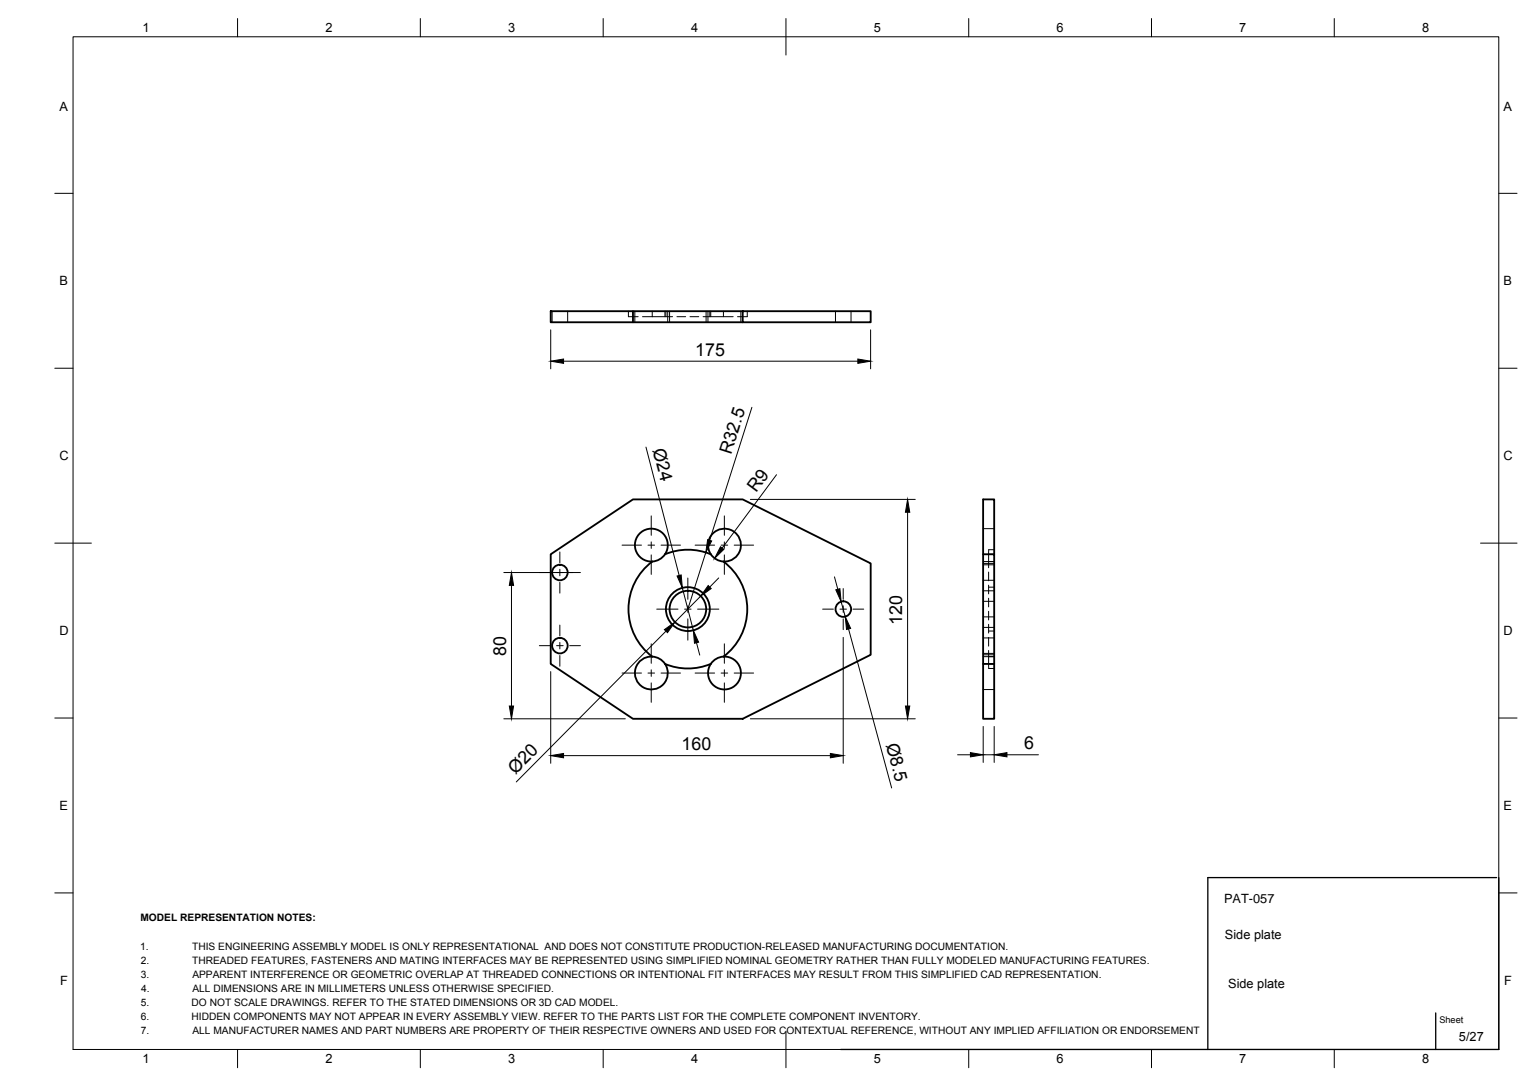
ISO-10303-21;
HEADER;
/* Generated by software containing ST-Developer
 * from STEP Tools, Inc. (www.steptools.com) 
 */

FILE_DESCRIPTION(
/* description */ ('Bearing-mounted hook block'),
/* implementation_level */ '2;1');

FILE_NAME(
/* name */ 'Side plate.step',
/* time_stamp */ '2026-10-28T22:30:11-07:00',
/* author */ (''),
/* organization */ (''),
/* preprocessor_version */ 'ST-DEVELOPER v20.2',
/* originating_system */ 'Autodesk Translation Framework v15.17.0.0',
/* authorisation */ '');

FILE_SCHEMA (('AUTOMOTIVE_DESIGN { 1 0 10303 214 3 1 1 }'));
ENDSEC;

DATA;
#10=MECHANICAL_DESIGN_GEOMETRIC_PRESENTATION_REPRESENTATION('',(#323),#7609);
#275=SHAPE_REPRESENTATION_RELATIONSHIP('SRR','None',#7722,#299);
#299=ADVANCED_BREP_SHAPE_REPRESENTATION('',(#355),#7582);
#323=STYLED_ITEM('',(#7924),#355);
#355=MANIFOLD_SOLID_BREP('Body1',#3919);
#384=LINE('',#6087,#614);
#385=LINE('',#6089,#615);
#386=LINE('',#6093,#616);
#387=LINE('',#6096,#617);
#388=LINE('',#6099,#618);
#389=LINE('',#6101,#619);
#390=LINE('',#6105,#620);
#391=LINE('',#6109,#621);
#392=LINE('',#6112,#622);
#393=LINE('',#6117,#623);
#394=LINE('',#6124,#624);
#395=LINE('',#6131,#625);
#396=LINE('',#6141,#626);
#397=LINE('',#6148,#627);
#398=LINE('',#6154,#628);
#399=LINE('',#6160,#629);
#400=LINE('',#6165,#630);
#401=LINE('',#6169,#631);
#402=LINE('',#6171,#632);
#403=LINE('',#6173,#633);
#404=LINE('',#6174,#634);
#405=LINE('',#6177,#635);
#406=LINE('',#6179,#636);
#407=LINE('',#6180,#637);
#408=LINE('',#6183,#638);
#409=LINE('',#6185,#639);
#410=LINE('',#6186,#640);
#411=LINE('',#6189,#641);
#412=LINE('',#6191,#642);
#413=LINE('',#6192,#643);
#414=LINE('',#6195,#644);
#415=LINE('',#6197,#645);
#416=LINE('',#6198,#646);
#417=LINE('',#6201,#647);
#418=LINE('',#6203,#648);
#419=LINE('',#6204,#649);
#420=LINE('',#6207,#650);
#421=LINE('',#6209,#651);
#422=LINE('',#6210,#652);
#423=LINE('',#6212,#653);
#424=LINE('',#6213,#654);
#614=VECTOR('',#4785,1.);
#615=VECTOR('',#4786,1.);
#616=VECTOR('',#4791,1.);
#617=VECTOR('',#4794,1.);
#618=VECTOR('',#4797,1.);
#619=VECTOR('',#4798,1.);
#620=VECTOR('',#4803,1.2);
#621=VECTOR('',#4808,1.);
#622=VECTOR('',#4811,1.);
#623=VECTOR('',#4816,0.9);
#624=VECTOR('',#4825,0.9);
#625=VECTOR('',#4834,0.9);
#626=VECTOR('',#4847,0.9);
#627=VECTOR('',#4856,0.425);
#628=VECTOR('',#4863,0.425);
#629=VECTOR('',#4870,0.425);
#630=VECTOR('',#4877,1.);
#631=VECTOR('',#4880,1.);
#632=VECTOR('',#4881,1.);
#633=VECTOR('',#4882,1.);
#634=VECTOR('',#4883,1.);
#635=VECTOR('',#4886,1.);
#636=VECTOR('',#4887,1.);
#637=VECTOR('',#4888,1.);
#638=VECTOR('',#4891,1.);
#639=VECTOR('',#4892,1.);
#640=VECTOR('',#4893,1.);
#641=VECTOR('',#4896,1.);
#642=VECTOR('',#4897,1.);
#643=VECTOR('',#4898,1.);
#644=VECTOR('',#4901,1.);
#645=VECTOR('',#4902,1.);
#646=VECTOR('',#4903,1.);
#647=VECTOR('',#4906,1.);
#648=VECTOR('',#4907,1.);
#649=VECTOR('',#4908,1.);
#650=VECTOR('',#4911,1.);
#651=VECTOR('',#4912,1.);
#652=VECTOR('',#4913,1.);
#653=VECTOR('',#4916,1.);
#654=VECTOR('',#4917,1.);
#844=CYLINDRICAL_SURFACE('',#4232,3.25);
#845=CYLINDRICAL_SURFACE('',#4234,3.25);
#846=CYLINDRICAL_SURFACE('',#4236,3.25);
#847=CYLINDRICAL_SURFACE('',#4238,1.2);
#848=CYLINDRICAL_SURFACE('',#4240,3.25);
#849=CYLINDRICAL_SURFACE('',#4242,0.9);
#850=CYLINDRICAL_SURFACE('',#4246,0.9);
#851=CYLINDRICAL_SURFACE('',#4250,0.9);
#852=CYLINDRICAL_SURFACE('',#4256,0.9);
#853=CYLINDRICAL_SURFACE('',#4260,0.425);
#854=CYLINDRICAL_SURFACE('',#4263,0.425);
#855=CYLINDRICAL_SURFACE('',#4266,0.425);
#856=CYLINDRICAL_SURFACE('',#4269,1.);
#921=FACE_BOUND('',#1238,.T.);
#922=FACE_BOUND('',#1248,.T.);
#923=FACE_BOUND('',#1263,.T.);
#924=FACE_BOUND('',#1264,.T.);
#925=FACE_BOUND('',#1265,.T.);
#926=FACE_BOUND('',#1266,.T.);
#927=FACE_BOUND('',#1268,.T.);
#928=FACE_BOUND('',#1269,.T.);
#929=FACE_BOUND('',#1270,.T.);
#930=FACE_BOUND('',#1271,.T.);
#931=FACE_BOUND('',#1272,.T.);
#932=FACE_BOUND('',#1273,.T.);
#933=FACE_BOUND('',#1274,.T.);
#934=FACE_BOUND('',#1275,.T.);
#1001=FACE_OUTER_BOUND('',#1237,.T.);
#1002=FACE_OUTER_BOUND('',#1239,.T.);
#1003=FACE_OUTER_BOUND('',#1240,.T.);
#1004=FACE_OUTER_BOUND('',#1241,.T.);
#1005=FACE_OUTER_BOUND('',#1242,.T.);
#1006=FACE_OUTER_BOUND('',#1243,.T.);
#1007=FACE_OUTER_BOUND('',#1244,.T.);
#1008=FACE_OUTER_BOUND('',#1245,.T.);
#1009=FACE_OUTER_BOUND('',#1246,.T.);
#1010=FACE_OUTER_BOUND('',#1247,.T.);
#1011=FACE_OUTER_BOUND('',#1249,.T.);
#1012=FACE_OUTER_BOUND('',#1250,.T.);
#1013=FACE_OUTER_BOUND('',#1251,.T.);
#1014=FACE_OUTER_BOUND('',#1252,.T.);
#1015=FACE_OUTER_BOUND('',#1253,.T.);
#1016=FACE_OUTER_BOUND('',#1254,.T.);
#1017=FACE_OUTER_BOUND('',#1255,.T.);
#1018=FACE_OUTER_BOUND('',#1256,.T.);
#1019=FACE_OUTER_BOUND('',#1257,.T.);
#1020=FACE_OUTER_BOUND('',#1258,.T.);
#1021=FACE_OUTER_BOUND('',#1259,.T.);
#1022=FACE_OUTER_BOUND('',#1260,.T.);
#1023=FACE_OUTER_BOUND('',#1261,.T.);
#1024=FACE_OUTER_BOUND('',#1262,.T.);
#1025=FACE_OUTER_BOUND('',#1267,.T.);
#1237=EDGE_LOOP('',(#2590,#2591,#2592,#2593,#2594,#2595,#2596,#2597));
#1238=EDGE_LOOP('',(#2598));
#1239=EDGE_LOOP('',(#2599,#2600,#2601,#2602));
#1240=EDGE_LOOP('',(#2603,#2604,#2605,#2606));
#1241=EDGE_LOOP('',(#2607,#2608,#2609,#2610));
#1242=EDGE_LOOP('',(#2611,#2612,#2613,#2614));
#1243=EDGE_LOOP('',(#2615,#2616,#2617,#2618));
#1244=EDGE_LOOP('',(#2619,#2620,#2621,#2622,#2623,#2624,#2625,#2626));
#1245=EDGE_LOOP('',(#2627,#2628,#2629,#2630,#2631,#2632,#2633,#2634));
#1246=EDGE_LOOP('',(#2635,#2636,#2637,#2638,#2639,#2640,#2641,#2642));
#1247=EDGE_LOOP('',(#2643));
#1248=EDGE_LOOP('',(#2644));
#1249=EDGE_LOOP('',(#2645,#2646,#2647,#2648,#2649,#2650,#2651,#2652));
#1250=EDGE_LOOP('',(#2653,#2654,#2655,#2656));
#1251=EDGE_LOOP('',(#2657,#2658,#2659,#2660));
#1252=EDGE_LOOP('',(#2661,#2662,#2663,#2664));
#1253=EDGE_LOOP('',(#2665,#2666,#2667,#2668));
#1254=EDGE_LOOP('',(#2669,#2670,#2671,#2672));
#1255=EDGE_LOOP('',(#2673,#2674,#2675,#2676));
#1256=EDGE_LOOP('',(#2677,#2678,#2679,#2680));
#1257=EDGE_LOOP('',(#2681,#2682,#2683,#2684));
#1258=EDGE_LOOP('',(#2685,#2686,#2687,#2688));
#1259=EDGE_LOOP('',(#2689,#2690,#2691,#2692));
#1260=EDGE_LOOP('',(#2693,#2694,#2695,#2696));
#1261=EDGE_LOOP('',(#2697,#2698,#2699,#2700));
#1262=EDGE_LOOP('',(#2701,#2702,#2703,#2704,#2705,#2706,#2707,#2708));
#1263=EDGE_LOOP('',(#2709,#2710,#2711,#2712,#2713,#2714,#2715,#2716,#2717,
#2718,#2719,#2720));
#1264=EDGE_LOOP('',(#2721));
#1265=EDGE_LOOP('',(#2722));
#1266=EDGE_LOOP('',(#2723));
#1267=EDGE_LOOP('',(#2724,#2725,#2726,#2727,#2728,#2729,#2730,#2731));
#1268=EDGE_LOOP('',(#2732));
#1269=EDGE_LOOP('',(#2733));
#1270=EDGE_LOOP('',(#2734));
#1271=EDGE_LOOP('',(#2735));
#1272=EDGE_LOOP('',(#2736));
#1273=EDGE_LOOP('',(#2737));
#1274=EDGE_LOOP('',(#2738));
#1275=EDGE_LOOP('',(#2739));
#1553=CIRCLE('',#4223,0.9);
#1554=CIRCLE('',#4224,3.25);
#1555=CIRCLE('',#4225,0.9);
#1556=CIRCLE('',#4226,3.25);
#1557=CIRCLE('',#4227,0.9);
#1558=CIRCLE('',#4228,3.25);
#1559=CIRCLE('',#4229,0.9);
#1560=CIRCLE('',#4230,3.25);
#1561=CIRCLE('',#4231,1.2);
#1562=CIRCLE('',#4233,3.25);
#1563=CIRCLE('',#4235,3.25);
#1564=CIRCLE('',#4237,3.25);
#1565=CIRCLE('',#4239,1.2);
#1566=CIRCLE('',#4241,3.25);
#1567=CIRCLE('',#4243,0.9);
#1568=CIRCLE('',#4244,0.9);
#1569=CIRCLE('',#4245,0.9);
#1570=CIRCLE('',#4247,0.9);
#1571=CIRCLE('',#4248,0.9);
#1572=CIRCLE('',#4249,0.9);
#1573=CIRCLE('',#4251,0.9);
#1574=CIRCLE('',#4252,0.9);
#1575=CIRCLE('',#4253,0.9);
#1576=CIRCLE('',#4255,1.);
#1577=CIRCLE('',#4257,0.9);
#1578=CIRCLE('',#4258,0.9);
#1579=CIRCLE('',#4259,0.9);
#1580=CIRCLE('',#4261,0.425);
#1581=CIRCLE('',#4262,0.425);
#1582=CIRCLE('',#4264,0.425);
#1583=CIRCLE('',#4265,0.425);
#1584=CIRCLE('',#4267,0.425);
#1585=CIRCLE('',#4268,0.425);
#1586=CIRCLE('',#4270,1.);
#1778=VERTEX_POINT('',#6067);
#1779=VERTEX_POINT('',#6068);
#1780=VERTEX_POINT('',#6070);
#1781=VERTEX_POINT('',#6072);
#1782=VERTEX_POINT('',#6074);
#1783=VERTEX_POINT('',#6076);
#1784=VERTEX_POINT('',#6078);
#1785=VERTEX_POINT('',#6080);
#1786=VERTEX_POINT('',#6083);
#1787=VERTEX_POINT('',#6086);
#1788=VERTEX_POINT('',#6088);
#1789=VERTEX_POINT('',#6092);
#1790=VERTEX_POINT('',#6094);
#1791=VERTEX_POINT('',#6098);
#1792=VERTEX_POINT('',#6100);
#1793=VERTEX_POINT('',#6104);
#1794=VERTEX_POINT('',#6108);
#1795=VERTEX_POINT('',#6110);
#1796=VERTEX_POINT('',#6114);
#1797=VERTEX_POINT('',#6116);
#1798=VERTEX_POINT('',#6121);
#1799=VERTEX_POINT('',#6123);
#1800=VERTEX_POINT('',#6128);
#1801=VERTEX_POINT('',#6130);
#1802=VERTEX_POINT('',#6135);
#1803=VERTEX_POINT('',#6138);
#1804=VERTEX_POINT('',#6140);
#1805=VERTEX_POINT('',#6145);
#1806=VERTEX_POINT('',#6147);
#1807=VERTEX_POINT('',#6151);
#1808=VERTEX_POINT('',#6153);
#1809=VERTEX_POINT('',#6157);
#1810=VERTEX_POINT('',#6159);
#1811=VERTEX_POINT('',#6163);
#1812=VERTEX_POINT('',#6167);
#1813=VERTEX_POINT('',#6168);
#1814=VERTEX_POINT('',#6170);
#1815=VERTEX_POINT('',#6172);
#1816=VERTEX_POINT('',#6176);
#1817=VERTEX_POINT('',#6178);
#1818=VERTEX_POINT('',#6182);
#1819=VERTEX_POINT('',#6184);
#1820=VERTEX_POINT('',#6188);
#1821=VERTEX_POINT('',#6190);
#1822=VERTEX_POINT('',#6194);
#1823=VERTEX_POINT('',#6196);
#1824=VERTEX_POINT('',#6200);
#1825=VERTEX_POINT('',#6202);
#1826=VERTEX_POINT('',#6206);
#1827=VERTEX_POINT('',#6208);
#2105=EDGE_CURVE('',#1778,#1779,#1553,.T.);
#2106=EDGE_CURVE('',#1778,#1780,#1554,.T.);
#2107=EDGE_CURVE('',#1781,#1780,#1555,.T.);
#2108=EDGE_CURVE('',#1781,#1782,#1556,.T.);
#2109=EDGE_CURVE('',#1783,#1782,#1557,.T.);
#2110=EDGE_CURVE('',#1783,#1784,#1558,.T.);
#2111=EDGE_CURVE('',#1785,#1784,#1559,.T.);
#2112=EDGE_CURVE('',#1785,#1779,#1560,.T.);
#2113=EDGE_CURVE('',#1786,#1786,#1561,.T.);
#2114=EDGE_CURVE('',#1784,#1787,#384,.T.);
#2115=EDGE_CURVE('',#1788,#1783,#385,.T.);
#2116=EDGE_CURVE('',#1787,#1788,#1562,.T.);
#2117=EDGE_CURVE('',#1789,#1781,#386,.T.);
#2118=EDGE_CURVE('',#1790,#1789,#1563,.T.);
#2119=EDGE_CURVE('',#1782,#1790,#387,.T.);
#2120=EDGE_CURVE('',#1779,#1791,#388,.T.);
#2121=EDGE_CURVE('',#1792,#1785,#389,.T.);
#2122=EDGE_CURVE('',#1791,#1792,#1564,.T.);
#2123=EDGE_CURVE('',#1786,#1793,#390,.T.);
#2124=EDGE_CURVE('',#1793,#1793,#1565,.T.);
#2125=EDGE_CURVE('',#1794,#1778,#391,.T.);
#2126=EDGE_CURVE('',#1795,#1794,#1566,.T.);
#2127=EDGE_CURVE('',#1780,#1795,#392,.T.);
#2128=EDGE_CURVE('',#1796,#1796,#1567,.T.);
#2129=EDGE_CURVE('',#1796,#1797,#393,.T.);
#2130=EDGE_CURVE('',#1794,#1797,#1568,.T.);
#2131=EDGE_CURVE('',#1797,#1791,#1569,.T.);
#2132=EDGE_CURVE('',#1798,#1798,#1570,.T.);
#2133=EDGE_CURVE('',#1798,#1799,#394,.T.);
#2134=EDGE_CURVE('',#1792,#1799,#1571,.T.);
#2135=EDGE_CURVE('',#1799,#1787,#1572,.T.);
#2136=EDGE_CURVE('',#1800,#1800,#1573,.T.);
#2137=EDGE_CURVE('',#1800,#1801,#395,.T.);
#2138=EDGE_CURVE('',#1788,#1801,#1574,.T.);
#2139=EDGE_CURVE('',#1801,#1790,#1575,.T.);
#2140=EDGE_CURVE('',#1802,#1802,#1576,.T.);
#2141=EDGE_CURVE('',#1803,#1803,#1577,.T.);
#2142=EDGE_CURVE('',#1803,#1804,#396,.T.);
#2143=EDGE_CURVE('',#1789,#1804,#1578,.T.);
#2144=EDGE_CURVE('',#1804,#1795,#1579,.T.);
#2145=EDGE_CURVE('',#1805,#1805,#1580,.T.);
#2146=EDGE_CURVE('',#1805,#1806,#397,.T.);
#2147=EDGE_CURVE('',#1806,#1806,#1581,.T.);
#2148=EDGE_CURVE('',#1807,#1807,#1582,.T.);
#2149=EDGE_CURVE('',#1807,#1808,#398,.T.);
#2150=EDGE_CURVE('',#1808,#1808,#1583,.T.);
#2151=EDGE_CURVE('',#1809,#1809,#1584,.T.);
#2152=EDGE_CURVE('',#1809,#1810,#399,.T.);
#2153=EDGE_CURVE('',#1810,#1810,#1585,.T.);
#2154=EDGE_CURVE('',#1811,#1811,#1586,.T.);
#2155=EDGE_CURVE('',#1811,#1802,#400,.T.);
#2156=EDGE_CURVE('',#1812,#1813,#401,.T.);
#2157=EDGE_CURVE('',#1812,#1814,#402,.T.);
#2158=EDGE_CURVE('',#1815,#1814,#403,.T.);
#2159=EDGE_CURVE('',#1813,#1815,#404,.T.);
#2160=EDGE_CURVE('',#1813,#1816,#405,.T.);
#2161=EDGE_CURVE('',#1817,#1815,#406,.T.);
#2162=EDGE_CURVE('',#1816,#1817,#407,.T.);
#2163=EDGE_CURVE('',#1816,#1818,#408,.T.);
#2164=EDGE_CURVE('',#1819,#1817,#409,.T.);
#2165=EDGE_CURVE('',#1818,#1819,#410,.T.);
#2166=EDGE_CURVE('',#1818,#1820,#411,.T.);
#2167=EDGE_CURVE('',#1821,#1819,#412,.T.);
#2168=EDGE_CURVE('',#1820,#1821,#413,.T.);
#2169=EDGE_CURVE('',#1820,#1822,#414,.T.);
#2170=EDGE_CURVE('',#1823,#1821,#415,.T.);
#2171=EDGE_CURVE('',#1822,#1823,#416,.T.);
#2172=EDGE_CURVE('',#1822,#1824,#417,.T.);
#2173=EDGE_CURVE('',#1825,#1823,#418,.T.);
#2174=EDGE_CURVE('',#1824,#1825,#419,.T.);
#2175=EDGE_CURVE('',#1824,#1826,#420,.T.);
#2176=EDGE_CURVE('',#1827,#1825,#421,.T.);
#2177=EDGE_CURVE('',#1826,#1827,#422,.T.);
#2178=EDGE_CURVE('',#1826,#1812,#423,.T.);
#2179=EDGE_CURVE('',#1814,#1827,#424,.T.);
#2590=ORIENTED_EDGE('',*,*,#2105,.F.);
#2591=ORIENTED_EDGE('',*,*,#2106,.T.);
#2592=ORIENTED_EDGE('',*,*,#2107,.F.);
#2593=ORIENTED_EDGE('',*,*,#2108,.T.);
#2594=ORIENTED_EDGE('',*,*,#2109,.F.);
#2595=ORIENTED_EDGE('',*,*,#2110,.T.);
#2596=ORIENTED_EDGE('',*,*,#2111,.F.);
#2597=ORIENTED_EDGE('',*,*,#2112,.T.);
#2598=ORIENTED_EDGE('',*,*,#2113,.T.);
#2599=ORIENTED_EDGE('',*,*,#2114,.F.);
#2600=ORIENTED_EDGE('',*,*,#2110,.F.);
#2601=ORIENTED_EDGE('',*,*,#2115,.F.);
#2602=ORIENTED_EDGE('',*,*,#2116,.F.);
#2603=ORIENTED_EDGE('',*,*,#2117,.F.);
#2604=ORIENTED_EDGE('',*,*,#2118,.F.);
#2605=ORIENTED_EDGE('',*,*,#2119,.F.);
#2606=ORIENTED_EDGE('',*,*,#2108,.F.);
#2607=ORIENTED_EDGE('',*,*,#2120,.F.);
#2608=ORIENTED_EDGE('',*,*,#2112,.F.);
#2609=ORIENTED_EDGE('',*,*,#2121,.F.);
#2610=ORIENTED_EDGE('',*,*,#2122,.F.);
#2611=ORIENTED_EDGE('',*,*,#2113,.F.);
#2612=ORIENTED_EDGE('',*,*,#2123,.T.);
#2613=ORIENTED_EDGE('',*,*,#2124,.F.);
#2614=ORIENTED_EDGE('',*,*,#2123,.F.);
#2615=ORIENTED_EDGE('',*,*,#2125,.F.);
#2616=ORIENTED_EDGE('',*,*,#2126,.F.);
#2617=ORIENTED_EDGE('',*,*,#2127,.F.);
#2618=ORIENTED_EDGE('',*,*,#2106,.F.);
#2619=ORIENTED_EDGE('',*,*,#2128,.F.);
#2620=ORIENTED_EDGE('',*,*,#2129,.T.);
#2621=ORIENTED_EDGE('',*,*,#2130,.F.);
#2622=ORIENTED_EDGE('',*,*,#2125,.T.);
#2623=ORIENTED_EDGE('',*,*,#2105,.T.);
#2624=ORIENTED_EDGE('',*,*,#2120,.T.);
#2625=ORIENTED_EDGE('',*,*,#2131,.F.);
#2626=ORIENTED_EDGE('',*,*,#2129,.F.);
#2627=ORIENTED_EDGE('',*,*,#2132,.F.);
#2628=ORIENTED_EDGE('',*,*,#2133,.T.);
#2629=ORIENTED_EDGE('',*,*,#2134,.F.);
#2630=ORIENTED_EDGE('',*,*,#2121,.T.);
#2631=ORIENTED_EDGE('',*,*,#2111,.T.);
#2632=ORIENTED_EDGE('',*,*,#2114,.T.);
#2633=ORIENTED_EDGE('',*,*,#2135,.F.);
#2634=ORIENTED_EDGE('',*,*,#2133,.F.);
#2635=ORIENTED_EDGE('',*,*,#2136,.F.);
#2636=ORIENTED_EDGE('',*,*,#2137,.T.);
#2637=ORIENTED_EDGE('',*,*,#2138,.F.);
#2638=ORIENTED_EDGE('',*,*,#2115,.T.);
#2639=ORIENTED_EDGE('',*,*,#2109,.T.);
#2640=ORIENTED_EDGE('',*,*,#2119,.T.);
#2641=ORIENTED_EDGE('',*,*,#2139,.F.);
#2642=ORIENTED_EDGE('',*,*,#2137,.F.);
#2643=ORIENTED_EDGE('',*,*,#2124,.T.);
#2644=ORIENTED_EDGE('',*,*,#2140,.T.);
#2645=ORIENTED_EDGE('',*,*,#2141,.F.);
#2646=ORIENTED_EDGE('',*,*,#2142,.T.);
#2647=ORIENTED_EDGE('',*,*,#2143,.F.);
#2648=ORIENTED_EDGE('',*,*,#2117,.T.);
#2649=ORIENTED_EDGE('',*,*,#2107,.T.);
#2650=ORIENTED_EDGE('',*,*,#2127,.T.);
#2651=ORIENTED_EDGE('',*,*,#2144,.F.);
#2652=ORIENTED_EDGE('',*,*,#2142,.F.);
#2653=ORIENTED_EDGE('',*,*,#2145,.F.);
#2654=ORIENTED_EDGE('',*,*,#2146,.T.);
#2655=ORIENTED_EDGE('',*,*,#2147,.F.);
#2656=ORIENTED_EDGE('',*,*,#2146,.F.);
#2657=ORIENTED_EDGE('',*,*,#2148,.F.);
#2658=ORIENTED_EDGE('',*,*,#2149,.T.);
#2659=ORIENTED_EDGE('',*,*,#2150,.F.);
#2660=ORIENTED_EDGE('',*,*,#2149,.F.);
#2661=ORIENTED_EDGE('',*,*,#2151,.F.);
#2662=ORIENTED_EDGE('',*,*,#2152,.T.);
#2663=ORIENTED_EDGE('',*,*,#2153,.F.);
#2664=ORIENTED_EDGE('',*,*,#2152,.F.);
#2665=ORIENTED_EDGE('',*,*,#2154,.F.);
#2666=ORIENTED_EDGE('',*,*,#2155,.T.);
#2667=ORIENTED_EDGE('',*,*,#2140,.F.);
#2668=ORIENTED_EDGE('',*,*,#2155,.F.);
#2669=ORIENTED_EDGE('',*,*,#2156,.F.);
#2670=ORIENTED_EDGE('',*,*,#2157,.T.);
#2671=ORIENTED_EDGE('',*,*,#2158,.F.);
#2672=ORIENTED_EDGE('',*,*,#2159,.F.);
#2673=ORIENTED_EDGE('',*,*,#2160,.F.);
#2674=ORIENTED_EDGE('',*,*,#2159,.T.);
#2675=ORIENTED_EDGE('',*,*,#2161,.F.);
#2676=ORIENTED_EDGE('',*,*,#2162,.F.);
#2677=ORIENTED_EDGE('',*,*,#2163,.F.);
#2678=ORIENTED_EDGE('',*,*,#2162,.T.);
#2679=ORIENTED_EDGE('',*,*,#2164,.F.);
#2680=ORIENTED_EDGE('',*,*,#2165,.F.);
#2681=ORIENTED_EDGE('',*,*,#2166,.F.);
#2682=ORIENTED_EDGE('',*,*,#2165,.T.);
#2683=ORIENTED_EDGE('',*,*,#2167,.F.);
#2684=ORIENTED_EDGE('',*,*,#2168,.F.);
#2685=ORIENTED_EDGE('',*,*,#2169,.F.);
#2686=ORIENTED_EDGE('',*,*,#2168,.T.);
#2687=ORIENTED_EDGE('',*,*,#2170,.F.);
#2688=ORIENTED_EDGE('',*,*,#2171,.F.);
#2689=ORIENTED_EDGE('',*,*,#2172,.F.);
#2690=ORIENTED_EDGE('',*,*,#2171,.T.);
#2691=ORIENTED_EDGE('',*,*,#2173,.F.);
#2692=ORIENTED_EDGE('',*,*,#2174,.F.);
#2693=ORIENTED_EDGE('',*,*,#2175,.F.);
#2694=ORIENTED_EDGE('',*,*,#2174,.T.);
#2695=ORIENTED_EDGE('',*,*,#2176,.F.);
#2696=ORIENTED_EDGE('',*,*,#2177,.F.);
#2697=ORIENTED_EDGE('',*,*,#2178,.F.);
#2698=ORIENTED_EDGE('',*,*,#2177,.T.);
#2699=ORIENTED_EDGE('',*,*,#2179,.F.);
#2700=ORIENTED_EDGE('',*,*,#2157,.F.);
#2701=ORIENTED_EDGE('',*,*,#2179,.T.);
#2702=ORIENTED_EDGE('',*,*,#2176,.T.);
#2703=ORIENTED_EDGE('',*,*,#2173,.T.);
#2704=ORIENTED_EDGE('',*,*,#2170,.T.);
#2705=ORIENTED_EDGE('',*,*,#2167,.T.);
#2706=ORIENTED_EDGE('',*,*,#2164,.T.);
#2707=ORIENTED_EDGE('',*,*,#2161,.T.);
#2708=ORIENTED_EDGE('',*,*,#2158,.T.);
#2709=ORIENTED_EDGE('',*,*,#2126,.T.);
#2710=ORIENTED_EDGE('',*,*,#2130,.T.);
#2711=ORIENTED_EDGE('',*,*,#2131,.T.);
#2712=ORIENTED_EDGE('',*,*,#2122,.T.);
#2713=ORIENTED_EDGE('',*,*,#2134,.T.);
#2714=ORIENTED_EDGE('',*,*,#2135,.T.);
#2715=ORIENTED_EDGE('',*,*,#2116,.T.);
#2716=ORIENTED_EDGE('',*,*,#2138,.T.);
#2717=ORIENTED_EDGE('',*,*,#2139,.T.);
#2718=ORIENTED_EDGE('',*,*,#2118,.T.);
#2719=ORIENTED_EDGE('',*,*,#2143,.T.);
#2720=ORIENTED_EDGE('',*,*,#2144,.T.);
#2721=ORIENTED_EDGE('',*,*,#2153,.T.);
#2722=ORIENTED_EDGE('',*,*,#2150,.T.);
#2723=ORIENTED_EDGE('',*,*,#2147,.T.);
#2724=ORIENTED_EDGE('',*,*,#2178,.T.);
#2725=ORIENTED_EDGE('',*,*,#2156,.T.);
#2726=ORIENTED_EDGE('',*,*,#2160,.T.);
#2727=ORIENTED_EDGE('',*,*,#2163,.T.);
#2728=ORIENTED_EDGE('',*,*,#2166,.T.);
#2729=ORIENTED_EDGE('',*,*,#2169,.T.);
#2730=ORIENTED_EDGE('',*,*,#2172,.T.);
#2731=ORIENTED_EDGE('',*,*,#2175,.T.);
#2732=ORIENTED_EDGE('',*,*,#2154,.T.);
#2733=ORIENTED_EDGE('',*,*,#2151,.T.);
#2734=ORIENTED_EDGE('',*,*,#2148,.T.);
#2735=ORIENTED_EDGE('',*,*,#2145,.T.);
#2736=ORIENTED_EDGE('',*,*,#2136,.T.);
#2737=ORIENTED_EDGE('',*,*,#2128,.T.);
#2738=ORIENTED_EDGE('',*,*,#2141,.T.);
#2739=ORIENTED_EDGE('',*,*,#2132,.T.);
#3560=PLANE('',#4222);
#3561=PLANE('',#4254);
#3562=PLANE('',#4271);
#3563=PLANE('',#4272);
#3564=PLANE('',#4273);
#3565=PLANE('',#4274);
#3566=PLANE('',#4275);
#3567=PLANE('',#4276);
#3568=PLANE('',#4277);
#3569=PLANE('',#4278);
#3570=PLANE('',#4279);
#3571=PLANE('',#4280);
#3683=ADVANCED_FACE('',(#1001,#921),#3560,.T.);
#3684=ADVANCED_FACE('',(#1002),#844,.F.);
#3685=ADVANCED_FACE('',(#1003),#845,.F.);
#3686=ADVANCED_FACE('',(#1004),#846,.F.);
#3687=ADVANCED_FACE('',(#1005),#847,.T.);
#3688=ADVANCED_FACE('',(#1006),#848,.F.);
#3689=ADVANCED_FACE('',(#1007),#849,.F.);
#3690=ADVANCED_FACE('',(#1008),#850,.F.);
#3691=ADVANCED_FACE('',(#1009),#851,.F.);
#3692=ADVANCED_FACE('',(#1010,#922),#3561,.T.);
#3693=ADVANCED_FACE('',(#1011),#852,.F.);
#3694=ADVANCED_FACE('',(#1012),#853,.F.);
#3695=ADVANCED_FACE('',(#1013),#854,.F.);
#3696=ADVANCED_FACE('',(#1014),#855,.F.);
#3697=ADVANCED_FACE('',(#1015),#856,.F.);
#3698=ADVANCED_FACE('',(#1016),#3562,.T.);
#3699=ADVANCED_FACE('',(#1017),#3563,.T.);
#3700=ADVANCED_FACE('',(#1018),#3564,.T.);
#3701=ADVANCED_FACE('',(#1019),#3565,.T.);
#3702=ADVANCED_FACE('',(#1020),#3566,.T.);
#3703=ADVANCED_FACE('',(#1021),#3567,.T.);
#3704=ADVANCED_FACE('',(#1022),#3568,.T.);
#3705=ADVANCED_FACE('',(#1023),#3569,.T.);
#3706=ADVANCED_FACE('',(#1024,#923,#924,#925,#926),#3570,.T.);
#3707=ADVANCED_FACE('',(#1025,#927,#928,#929,#930,#931,#932,#933,#934),
#3571,.F.);
#3919=CLOSED_SHELL('',(#3683,#3684,#3685,#3686,#3687,#3688,#3689,#3690,
#3691,#3692,#3693,#3694,#3695,#3696,#3697,#3698,#3699,#3700,#3701,#3702,
#3703,#3704,#3705,#3706,#3707));
#4221=AXIS2_PLACEMENT_3D('',#6065,#4761,#4762);
#4222=AXIS2_PLACEMENT_3D('',#6066,#4763,#4764);
#4223=AXIS2_PLACEMENT_3D('',#6069,#4765,#4766);
#4224=AXIS2_PLACEMENT_3D('',#6071,#4767,#4768);
#4225=AXIS2_PLACEMENT_3D('',#6073,#4769,#4770);
#4226=AXIS2_PLACEMENT_3D('',#6075,#4771,#4772);
#4227=AXIS2_PLACEMENT_3D('',#6077,#4773,#4774);
#4228=AXIS2_PLACEMENT_3D('',#6079,#4775,#4776);
#4229=AXIS2_PLACEMENT_3D('',#6081,#4777,#4778);
#4230=AXIS2_PLACEMENT_3D('',#6082,#4779,#4780);
#4231=AXIS2_PLACEMENT_3D('',#6084,#4781,#4782);
#4232=AXIS2_PLACEMENT_3D('',#6085,#4783,#4784);
#4233=AXIS2_PLACEMENT_3D('',#6090,#4787,#4788);
#4234=AXIS2_PLACEMENT_3D('',#6091,#4789,#4790);
#4235=AXIS2_PLACEMENT_3D('',#6095,#4792,#4793);
#4236=AXIS2_PLACEMENT_3D('',#6097,#4795,#4796);
#4237=AXIS2_PLACEMENT_3D('',#6102,#4799,#4800);
#4238=AXIS2_PLACEMENT_3D('',#6103,#4801,#4802);
#4239=AXIS2_PLACEMENT_3D('',#6106,#4804,#4805);
#4240=AXIS2_PLACEMENT_3D('',#6107,#4806,#4807);
#4241=AXIS2_PLACEMENT_3D('',#6111,#4809,#4810);
#4242=AXIS2_PLACEMENT_3D('',#6113,#4812,#4813);
#4243=AXIS2_PLACEMENT_3D('',#6115,#4814,#4815);
#4244=AXIS2_PLACEMENT_3D('',#6118,#4817,#4818);
#4245=AXIS2_PLACEMENT_3D('',#6119,#4819,#4820);
#4246=AXIS2_PLACEMENT_3D('',#6120,#4821,#4822);
#4247=AXIS2_PLACEMENT_3D('',#6122,#4823,#4824);
#4248=AXIS2_PLACEMENT_3D('',#6125,#4826,#4827);
#4249=AXIS2_PLACEMENT_3D('',#6126,#4828,#4829);
#4250=AXIS2_PLACEMENT_3D('',#6127,#4830,#4831);
#4251=AXIS2_PLACEMENT_3D('',#6129,#4832,#4833);
#4252=AXIS2_PLACEMENT_3D('',#6132,#4835,#4836);
#4253=AXIS2_PLACEMENT_3D('',#6133,#4837,#4838);
#4254=AXIS2_PLACEMENT_3D('',#6134,#4839,#4840);
#4255=AXIS2_PLACEMENT_3D('',#6136,#4841,#4842);
#4256=AXIS2_PLACEMENT_3D('',#6137,#4843,#4844);
#4257=AXIS2_PLACEMENT_3D('',#6139,#4845,#4846);
#4258=AXIS2_PLACEMENT_3D('',#6142,#4848,#4849);
#4259=AXIS2_PLACEMENT_3D('',#6143,#4850,#4851);
#4260=AXIS2_PLACEMENT_3D('',#6144,#4852,#4853);
#4261=AXIS2_PLACEMENT_3D('',#6146,#4854,#4855);
#4262=AXIS2_PLACEMENT_3D('',#6149,#4857,#4858);
#4263=AXIS2_PLACEMENT_3D('',#6150,#4859,#4860);
#4264=AXIS2_PLACEMENT_3D('',#6152,#4861,#4862);
#4265=AXIS2_PLACEMENT_3D('',#6155,#4864,#4865);
#4266=AXIS2_PLACEMENT_3D('',#6156,#4866,#4867);
#4267=AXIS2_PLACEMENT_3D('',#6158,#4868,#4869);
#4268=AXIS2_PLACEMENT_3D('',#6161,#4871,#4872);
#4269=AXIS2_PLACEMENT_3D('',#6162,#4873,#4874);
#4270=AXIS2_PLACEMENT_3D('',#6164,#4875,#4876);
#4271=AXIS2_PLACEMENT_3D('',#6166,#4878,#4879);
#4272=AXIS2_PLACEMENT_3D('',#6175,#4884,#4885);
#4273=AXIS2_PLACEMENT_3D('',#6181,#4889,#4890);
#4274=AXIS2_PLACEMENT_3D('',#6187,#4894,#4895);
#4275=AXIS2_PLACEMENT_3D('',#6193,#4899,#4900);
#4276=AXIS2_PLACEMENT_3D('',#6199,#4904,#4905);
#4277=AXIS2_PLACEMENT_3D('',#6205,#4909,#4910);
#4278=AXIS2_PLACEMENT_3D('',#6211,#4914,#4915);
#4279=AXIS2_PLACEMENT_3D('',#6214,#4918,#4919);
#4280=AXIS2_PLACEMENT_3D('',#6215,#4920,#4921);
#4761=DIRECTION('axis',(0.,0.,1.));
#4762=DIRECTION('refdir',(1.,0.,0.));
#4763=DIRECTION('center_axis',(0.,1.,0.));
#4764=DIRECTION('ref_axis',(1.,0.,0.));
#4765=DIRECTION('center_axis',(0.,1.,0.));
#4766=DIRECTION('ref_axis',(1.,0.,0.));
#4767=DIRECTION('center_axis',(0.,1.,0.));
#4768=DIRECTION('ref_axis',(1.,0.,0.));
#4769=DIRECTION('center_axis',(0.,1.,0.));
#4770=DIRECTION('ref_axis',(1.,0.,0.));
#4771=DIRECTION('center_axis',(0.,1.,0.));
#4772=DIRECTION('ref_axis',(1.,0.,0.));
#4773=DIRECTION('center_axis',(0.,1.,0.));
#4774=DIRECTION('ref_axis',(1.,0.,0.));
#4775=DIRECTION('center_axis',(0.,1.,0.));
#4776=DIRECTION('ref_axis',(1.,0.,0.));
#4777=DIRECTION('center_axis',(0.,1.,0.));
#4778=DIRECTION('ref_axis',(1.,0.,0.));
#4779=DIRECTION('center_axis',(0.,1.,0.));
#4780=DIRECTION('ref_axis',(1.,0.,0.));
#4781=DIRECTION('center_axis',(0.,-1.,0.));
#4782=DIRECTION('ref_axis',(1.,0.,0.));
#4783=DIRECTION('center_axis',(0.,1.,0.));
#4784=DIRECTION('ref_axis',(1.,0.,0.));
#4785=DIRECTION('',(0.,1.,0.));
#4786=DIRECTION('',(0.,-1.,0.));
#4787=DIRECTION('center_axis',(0.,-1.,0.));
#4788=DIRECTION('ref_axis',(1.,0.,0.));
#4789=DIRECTION('center_axis',(0.,1.,0.));
#4790=DIRECTION('ref_axis',(1.,0.,0.));
#4791=DIRECTION('',(0.,-1.,0.));
#4792=DIRECTION('center_axis',(0.,-1.,0.));
#4793=DIRECTION('ref_axis',(1.,0.,0.));
#4794=DIRECTION('',(0.,1.,0.));
#4795=DIRECTION('center_axis',(0.,1.,0.));
#4796=DIRECTION('ref_axis',(1.,0.,0.));
#4797=DIRECTION('',(0.,1.,0.));
#4798=DIRECTION('',(0.,-1.,0.));
#4799=DIRECTION('center_axis',(0.,-1.,0.));
#4800=DIRECTION('ref_axis',(1.,0.,0.));
#4801=DIRECTION('center_axis',(0.,1.,0.));
#4802=DIRECTION('ref_axis',(1.,0.,0.));
#4803=DIRECTION('',(0.,1.,0.));
#4804=DIRECTION('center_axis',(0.,1.,0.));
#4805=DIRECTION('ref_axis',(1.,0.,0.));
#4806=DIRECTION('center_axis',(0.,1.,0.));
#4807=DIRECTION('ref_axis',(-1.,0.,-1.22464679914735E-16));
#4808=DIRECTION('',(0.,-1.,0.));
#4809=DIRECTION('center_axis',(0.,-1.,0.));
#4810=DIRECTION('ref_axis',(1.,0.,0.));
#4811=DIRECTION('',(0.,1.,0.));
#4812=DIRECTION('center_axis',(0.,1.,0.));
#4813=DIRECTION('ref_axis',(1.,0.,0.));
#4814=DIRECTION('center_axis',(0.,1.,0.));
#4815=DIRECTION('ref_axis',(1.,0.,0.));
#4816=DIRECTION('',(0.,1.,0.));
#4817=DIRECTION('center_axis',(0.,-1.,0.));
#4818=DIRECTION('ref_axis',(1.,0.,0.));
#4819=DIRECTION('center_axis',(0.,-1.,0.));
#4820=DIRECTION('ref_axis',(1.,0.,0.));
#4821=DIRECTION('center_axis',(0.,1.,0.));
#4822=DIRECTION('ref_axis',(1.,0.,0.));
#4823=DIRECTION('center_axis',(0.,1.,0.));
#4824=DIRECTION('ref_axis',(1.,0.,0.));
#4825=DIRECTION('',(0.,1.,0.));
#4826=DIRECTION('center_axis',(0.,-1.,0.));
#4827=DIRECTION('ref_axis',(1.,0.,0.));
#4828=DIRECTION('center_axis',(0.,-1.,0.));
#4829=DIRECTION('ref_axis',(1.,0.,0.));
#4830=DIRECTION('center_axis',(0.,1.,0.));
#4831=DIRECTION('ref_axis',(1.,0.,0.));
#4832=DIRECTION('center_axis',(0.,1.,0.));
#4833=DIRECTION('ref_axis',(1.,0.,0.));
#4834=DIRECTION('',(0.,1.,0.));
#4835=DIRECTION('center_axis',(0.,-1.,0.));
#4836=DIRECTION('ref_axis',(1.,0.,0.));
#4837=DIRECTION('center_axis',(0.,-1.,0.));
#4838=DIRECTION('ref_axis',(1.,0.,0.));
#4839=DIRECTION('center_axis',(0.,1.,0.));
#4840=DIRECTION('ref_axis',(0.,0.,1.));
#4841=DIRECTION('center_axis',(0.,-1.,0.));
#4842=DIRECTION('ref_axis',(1.,0.,0.));
#4843=DIRECTION('center_axis',(0.,1.,0.));
#4844=DIRECTION('ref_axis',(1.,0.,0.));
#4845=DIRECTION('center_axis',(0.,1.,0.));
#4846=DIRECTION('ref_axis',(1.,0.,0.));
#4847=DIRECTION('',(0.,1.,0.));
#4848=DIRECTION('center_axis',(0.,-1.,0.));
#4849=DIRECTION('ref_axis',(1.,0.,0.));
#4850=DIRECTION('center_axis',(0.,-1.,0.));
#4851=DIRECTION('ref_axis',(1.,0.,0.));
#4852=DIRECTION('center_axis',(0.,1.,0.));
#4853=DIRECTION('ref_axis',(1.,0.,0.));
#4854=DIRECTION('center_axis',(0.,1.,0.));
#4855=DIRECTION('ref_axis',(1.,0.,0.));
#4856=DIRECTION('',(0.,1.,0.));
#4857=DIRECTION('center_axis',(0.,-1.,0.));
#4858=DIRECTION('ref_axis',(1.,0.,0.));
#4859=DIRECTION('center_axis',(0.,1.,0.));
#4860=DIRECTION('ref_axis',(1.,0.,0.));
#4861=DIRECTION('center_axis',(0.,1.,0.));
#4862=DIRECTION('ref_axis',(1.,0.,0.));
#4863=DIRECTION('',(0.,1.,0.));
#4864=DIRECTION('center_axis',(0.,-1.,0.));
#4865=DIRECTION('ref_axis',(1.,0.,0.));
#4866=DIRECTION('center_axis',(0.,1.,0.));
#4867=DIRECTION('ref_axis',(1.,0.,0.));
#4868=DIRECTION('center_axis',(0.,1.,0.));
#4869=DIRECTION('ref_axis',(1.,0.,0.));
#4870=DIRECTION('',(0.,1.,0.));
#4871=DIRECTION('center_axis',(0.,-1.,0.));
#4872=DIRECTION('ref_axis',(1.,0.,0.));
#4873=DIRECTION('center_axis',(0.,1.,0.));
#4874=DIRECTION('ref_axis',(1.,0.,0.));
#4875=DIRECTION('center_axis',(0.,1.,0.));
#4876=DIRECTION('ref_axis',(1.,0.,0.));
#4877=DIRECTION('',(0.,1.,0.));
#4878=DIRECTION('center_axis',(-0.832050294337844,0.,-0.554700196225229));
#4879=DIRECTION('ref_axis',(-0.554700196225229,0.,0.832050294337844));
#4880=DIRECTION('',(0.554700196225229,0.,-0.832050294337844));
#4881=DIRECTION('',(0.,1.,0.));
#4882=DIRECTION('',(-0.554700196225229,0.,0.832050294337844));
#4883=DIRECTION('',(0.,1.,0.));
#4884=DIRECTION('center_axis',(0.,0.,-1.));
#4885=DIRECTION('ref_axis',(-1.,0.,0.));
#4886=DIRECTION('',(1.,0.,0.));
#4887=DIRECTION('',(-1.,0.,0.));
#4888=DIRECTION('',(0.,1.,0.));
#4889=DIRECTION('center_axis',(0.832050294337844,0.,-0.554700196225229));
#4890=DIRECTION('ref_axis',(-0.554700196225229,0.,-0.832050294337844));
#4891=DIRECTION('',(0.554700196225229,0.,0.832050294337844));
#4892=DIRECTION('',(-0.554700196225229,0.,-0.832050294337844));
#4893=DIRECTION('',(0.,1.,0.));
#4894=DIRECTION('center_axis',(1.,0.,0.));
#4895=DIRECTION('ref_axis',(0.,0.,-1.));
#4896=DIRECTION('',(0.,0.,1.));
#4897=DIRECTION('',(0.,0.,-1.));
#4898=DIRECTION('',(0.,1.,0.));
#4899=DIRECTION('center_axis',(0.894427190999916,0.,0.447213595499958));
#4900=DIRECTION('ref_axis',(0.447213595499958,0.,-0.894427190999916));
#4901=DIRECTION('',(-0.447213595499958,0.,0.894427190999916));
#4902=DIRECTION('',(0.447213595499958,0.,-0.894427190999916));
#4903=DIRECTION('',(0.,1.,0.));
#4904=DIRECTION('center_axis',(0.,0.,1.));
#4905=DIRECTION('ref_axis',(1.,0.,0.));
#4906=DIRECTION('',(-1.,0.,0.));
#4907=DIRECTION('',(1.,0.,0.));
#4908=DIRECTION('',(0.,1.,0.));
#4909=DIRECTION('center_axis',(-0.894427190999916,0.,0.447213595499958));
#4910=DIRECTION('ref_axis',(0.447213595499958,0.,0.894427190999916));
#4911=DIRECTION('',(-0.447213595499958,0.,-0.894427190999916));
#4912=DIRECTION('',(0.447213595499958,0.,0.894427190999916));
#4913=DIRECTION('',(0.,1.,0.));
#4914=DIRECTION('center_axis',(-1.,0.,0.));
#4915=DIRECTION('ref_axis',(0.,0.,1.));
#4916=DIRECTION('',(0.,0.,-1.));
#4917=DIRECTION('',(0.,0.,1.));
#4918=DIRECTION('center_axis',(0.,1.,0.));
#4919=DIRECTION('ref_axis',(0.,0.,1.));
#4920=DIRECTION('center_axis',(0.,1.,0.));
#4921=DIRECTION('ref_axis',(1.,0.,0.));
#6065=CARTESIAN_POINT('',(0.,0.,0.));
#6066=CARTESIAN_POINT('Origin',(0.,-2.8,12.));
#6067=CARTESIAN_POINT('',(-2.99903459153175,-2.8,10.7476855351806));
#6068=CARTESIAN_POINT('',(-2.60150387000671,-2.8,10.0520067725117));
#6069=CARTESIAN_POINT('Origin',(-3.5,-2.8,10.));
#6070=CARTESIAN_POINT('',(-2.99903459153175,-2.8,13.2523144648194));
#6071=CARTESIAN_POINT('Origin',(0.,-2.8,12.));
#6072=CARTESIAN_POINT('',(-2.60150387000671,-2.8,13.9479932274883));
#6073=CARTESIAN_POINT('Origin',(-3.5,-2.8,14.));
#6074=CARTESIAN_POINT('',(2.60150387000671,-2.8,13.9479932274883));
#6075=CARTESIAN_POINT('Origin',(0.,-2.8,12.));
#6076=CARTESIAN_POINT('',(2.99903459153175,-2.8,13.2523144648194));
#6077=CARTESIAN_POINT('Origin',(3.5,-2.8,14.));
#6078=CARTESIAN_POINT('',(2.99903459153175,-2.8,10.7476855351806));
#6079=CARTESIAN_POINT('Origin',(0.,-2.8,12.));
#6080=CARTESIAN_POINT('',(2.60150387000671,-2.8,10.0520067725117));
#6081=CARTESIAN_POINT('Origin',(3.5,-2.8,10.));
#6082=CARTESIAN_POINT('Origin',(0.,-2.8,12.));
#6083=CARTESIAN_POINT('',(-1.2,-2.8,12.));
#6084=CARTESIAN_POINT('Origin',(0.,-2.8,12.));
#6085=CARTESIAN_POINT('Origin',(0.,-2.8,12.));
#6086=CARTESIAN_POINT('',(2.99903459153175,-2.5,10.7476855351806));
#6087=CARTESIAN_POINT('',(2.99903459153175,-2.8,10.7476855351806));
#6088=CARTESIAN_POINT('',(2.99903459153175,-2.5,13.2523144648194));
#6089=CARTESIAN_POINT('',(2.99903459153175,-2.8,13.2523144648194));
#6090=CARTESIAN_POINT('Origin',(0.,-2.5,12.));
#6091=CARTESIAN_POINT('Origin',(0.,-2.8,12.));
#6092=CARTESIAN_POINT('',(-2.60150387000671,-2.5,13.9479932274883));
#6093=CARTESIAN_POINT('',(-2.60150387000671,-2.8,13.9479932274883));
#6094=CARTESIAN_POINT('',(2.60150387000671,-2.5,13.9479932274883));
#6095=CARTESIAN_POINT('Origin',(0.,-2.5,12.));
#6096=CARTESIAN_POINT('',(2.60150387000671,-2.8,13.9479932274883));
#6097=CARTESIAN_POINT('Origin',(0.,-2.8,12.));
#6098=CARTESIAN_POINT('',(-2.60150387000671,-2.5,10.0520067725117));
#6099=CARTESIAN_POINT('',(-2.60150387000671,-2.8,10.0520067725117));
#6100=CARTESIAN_POINT('',(2.60150387000671,-2.5,10.0520067725117));
#6101=CARTESIAN_POINT('',(2.60150387000671,-2.8,10.0520067725117));
#6102=CARTESIAN_POINT('Origin',(0.,-2.5,12.));
#6103=CARTESIAN_POINT('Origin',(0.,-2.8,12.));
#6104=CARTESIAN_POINT('',(-1.2,-2.5,12.));
#6105=CARTESIAN_POINT('',(-1.2,-2.8,12.));
#6106=CARTESIAN_POINT('Origin',(0.,-2.5,12.));
#6107=CARTESIAN_POINT('Origin',(0.,-2.8,12.));
#6108=CARTESIAN_POINT('',(-2.99903459153175,-2.5,10.7476855351806));
#6109=CARTESIAN_POINT('',(-2.99903459153175,-2.8,10.7476855351806));
#6110=CARTESIAN_POINT('',(-2.99903459153175,-2.5,13.2523144648194));
#6111=CARTESIAN_POINT('Origin',(0.,-2.5,12.));
#6112=CARTESIAN_POINT('',(-2.99903459153175,-2.8,13.2523144648194));
#6113=CARTESIAN_POINT('Origin',(-3.5,-3.2,10.));
#6114=CARTESIAN_POINT('',(-4.4,-3.1,10.));
#6115=CARTESIAN_POINT('Origin',(-3.5,-3.1,10.));
#6116=CARTESIAN_POINT('',(-4.4,-2.5,10.));
#6117=CARTESIAN_POINT('',(-4.4,-3.2,10.));
#6118=CARTESIAN_POINT('Origin',(-3.5,-2.5,10.));
#6119=CARTESIAN_POINT('Origin',(-3.5,-2.5,10.));
#6120=CARTESIAN_POINT('Origin',(3.5,-3.2,10.));
#6121=CARTESIAN_POINT('',(2.6,-3.1,10.));
#6122=CARTESIAN_POINT('Origin',(3.5,-3.1,10.));
#6123=CARTESIAN_POINT('',(2.6,-2.5,10.));
#6124=CARTESIAN_POINT('',(2.6,-3.2,10.));
#6125=CARTESIAN_POINT('Origin',(3.5,-2.5,10.));
#6126=CARTESIAN_POINT('Origin',(3.5,-2.5,10.));
#6127=CARTESIAN_POINT('Origin',(3.5,-3.2,14.));
#6128=CARTESIAN_POINT('',(2.6,-3.1,14.));
#6129=CARTESIAN_POINT('Origin',(3.5,-3.1,14.));
#6130=CARTESIAN_POINT('',(2.6,-2.5,14.));
#6131=CARTESIAN_POINT('',(2.6,-3.2,14.));
#6132=CARTESIAN_POINT('Origin',(3.5,-2.5,14.));
#6133=CARTESIAN_POINT('Origin',(3.5,-2.5,14.));
#6134=CARTESIAN_POINT('Origin',(0.,-2.5,13.25));
#6135=CARTESIAN_POINT('',(-1.,-2.5,12.));
#6136=CARTESIAN_POINT('Origin',(0.,-2.5,12.));
#6137=CARTESIAN_POINT('Origin',(-3.5,-3.2,14.));
#6138=CARTESIAN_POINT('',(-4.4,-3.1,14.));
#6139=CARTESIAN_POINT('Origin',(-3.5,-3.1,14.));
#6140=CARTESIAN_POINT('',(-4.4,-2.5,14.));
#6141=CARTESIAN_POINT('',(-4.4,-3.2,14.));
#6142=CARTESIAN_POINT('Origin',(-3.5,-2.5,14.));
#6143=CARTESIAN_POINT('Origin',(-3.5,-2.5,14.));
#6144=CARTESIAN_POINT('Origin',(-2.,-3.2,5.));
#6145=CARTESIAN_POINT('',(-2.425,-3.1,5.));
#6146=CARTESIAN_POINT('Origin',(-2.,-3.1,5.));
#6147=CARTESIAN_POINT('',(-2.425,-2.5,5.));
#6148=CARTESIAN_POINT('',(-2.425,-3.2,5.));
#6149=CARTESIAN_POINT('Origin',(-2.,-2.5,5.));
#6150=CARTESIAN_POINT('Origin',(2.,-3.2,5.));
#6151=CARTESIAN_POINT('',(1.575,-3.1,5.));
#6152=CARTESIAN_POINT('Origin',(2.,-3.1,5.));
#6153=CARTESIAN_POINT('',(1.575,-2.5,5.));
#6154=CARTESIAN_POINT('',(1.575,-3.2,5.));
#6155=CARTESIAN_POINT('Origin',(2.,-2.5,5.));
#6156=CARTESIAN_POINT('Origin',(0.,-3.2,20.5));
#6157=CARTESIAN_POINT('',(-0.425,-3.1,20.5));
#6158=CARTESIAN_POINT('Origin',(0.,-3.1,20.5));
#6159=CARTESIAN_POINT('',(-0.425,-2.5,20.5));
#6160=CARTESIAN_POINT('',(-0.425,-3.2,20.5));
#6161=CARTESIAN_POINT('Origin',(0.,-2.5,20.5));
#6162=CARTESIAN_POINT('Origin',(0.,-3.2,12.));
#6163=CARTESIAN_POINT('',(-1.,-3.1,12.));
#6164=CARTESIAN_POINT('Origin',(0.,-3.1,12.));
#6165=CARTESIAN_POINT('',(-1.,-3.2,12.));
#6166=CARTESIAN_POINT('Origin',(-3.,-3.1,4.5));
#6167=CARTESIAN_POINT('',(-6.,-3.1,9.));
#6168=CARTESIAN_POINT('',(-3.,-3.1,4.5));
#6169=CARTESIAN_POINT('',(-6.,-3.1,9.));
#6170=CARTESIAN_POINT('',(-6.,-2.5,9.));
#6171=CARTESIAN_POINT('',(-6.,-3.1,9.));
#6172=CARTESIAN_POINT('',(-3.,-2.5,4.5));
#6173=CARTESIAN_POINT('',(-6.,-2.5,9.));
#6174=CARTESIAN_POINT('',(-3.,-3.1,4.5));
#6175=CARTESIAN_POINT('Origin',(3.,-3.1,4.5));
#6176=CARTESIAN_POINT('',(3.,-3.1,4.5));
#6177=CARTESIAN_POINT('',(-3.,-3.1,4.5));
#6178=CARTESIAN_POINT('',(3.,-2.5,4.5));
#6179=CARTESIAN_POINT('',(-3.,-2.5,4.5));
#6180=CARTESIAN_POINT('',(3.,-3.1,4.5));
#6181=CARTESIAN_POINT('Origin',(6.,-3.1,9.));
#6182=CARTESIAN_POINT('',(6.,-3.1,9.));
#6183=CARTESIAN_POINT('',(3.,-3.1,4.5));
#6184=CARTESIAN_POINT('',(6.,-2.5,9.));
#6185=CARTESIAN_POINT('',(3.,-2.5,4.5));
#6186=CARTESIAN_POINT('',(6.,-3.1,9.));
#6187=CARTESIAN_POINT('Origin',(6.,-3.1,15.));
#6188=CARTESIAN_POINT('',(6.,-3.1,15.));
#6189=CARTESIAN_POINT('',(6.,-3.1,9.));
#6190=CARTESIAN_POINT('',(6.,-2.5,15.));
#6191=CARTESIAN_POINT('',(6.,-2.5,9.));
#6192=CARTESIAN_POINT('',(6.,-3.1,15.));
#6193=CARTESIAN_POINT('Origin',(2.5,-3.1,22.));
#6194=CARTESIAN_POINT('',(2.5,-3.1,22.));
#6195=CARTESIAN_POINT('',(6.,-3.1,15.));
#6196=CARTESIAN_POINT('',(2.5,-2.5,22.));
#6197=CARTESIAN_POINT('',(6.,-2.5,15.));
#6198=CARTESIAN_POINT('',(2.5,-3.1,22.));
#6199=CARTESIAN_POINT('Origin',(-2.5,-3.1,22.));
#6200=CARTESIAN_POINT('',(-2.5,-3.1,22.));
#6201=CARTESIAN_POINT('',(2.5,-3.1,22.));
#6202=CARTESIAN_POINT('',(-2.5,-2.5,22.));
#6203=CARTESIAN_POINT('',(2.5,-2.5,22.));
#6204=CARTESIAN_POINT('',(-2.5,-3.1,22.));
#6205=CARTESIAN_POINT('Origin',(-6.,-3.1,15.));
#6206=CARTESIAN_POINT('',(-6.,-3.1,15.));
#6207=CARTESIAN_POINT('',(-2.5,-3.1,22.));
#6208=CARTESIAN_POINT('',(-6.,-2.5,15.));
#6209=CARTESIAN_POINT('',(-2.5,-2.5,22.));
#6210=CARTESIAN_POINT('',(-6.,-3.1,15.));
#6211=CARTESIAN_POINT('Origin',(-6.,-3.1,9.));
#6212=CARTESIAN_POINT('',(-6.,-3.1,15.));
#6213=CARTESIAN_POINT('',(-6.,-2.5,15.));
#6214=CARTESIAN_POINT('Origin',(0.,-2.5,13.25));
#6215=CARTESIAN_POINT('Origin',(0.,-3.1,13.25));
#7552=UNCERTAINTY_MEASURE_WITH_UNIT(LENGTH_MEASURE(0.001),#7610,
'DISTANCE_ACCURACY_VALUE',
'Maximum model space distance between geometric entities at asserted c
onnectivities');
#7579=UNCERTAINTY_MEASURE_WITH_UNIT(LENGTH_MEASURE(0.001),#7610,
'DISTANCE_ACCURACY_VALUE',
'Maximum model space distance between geometric entities at asserted c
onnectivities');
#7582=(
GEOMETRIC_REPRESENTATION_CONTEXT(3)
GLOBAL_UNCERTAINTY_ASSIGNED_CONTEXT((#7552))
GLOBAL_UNIT_ASSIGNED_CONTEXT((#7610,#7612,#7613))
REPRESENTATION_CONTEXT('','3D')
);
#7609=(
GEOMETRIC_REPRESENTATION_CONTEXT(3)
GLOBAL_UNCERTAINTY_ASSIGNED_CONTEXT((#7579))
GLOBAL_UNIT_ASSIGNED_CONTEXT((#7610,#7612,#7613))
REPRESENTATION_CONTEXT('','3D')
);
#7610=(
LENGTH_UNIT()
NAMED_UNIT(*)
SI_UNIT(.CENTI.,.METRE.)
);
#7612=(
NAMED_UNIT(*)
PLANE_ANGLE_UNIT()
SI_UNIT($,.RADIAN.)
);
#7613=(
NAMED_UNIT(*)
SI_UNIT($,.STERADIAN.)
SOLID_ANGLE_UNIT()
);
#7616=SHAPE_DEFINITION_REPRESENTATION(#7645,#7722);
#7645=PRODUCT_DEFINITION_SHAPE('',$,#7752);
#7722=SHAPE_REPRESENTATION('',(#4221),#7582);
#7749=PRODUCT_DEFINITION_CONTEXT('part definition',#7838,'design');
#7752=PRODUCT_DEFINITION('Side plate','Side plate',#7781,#7749);
#7781=PRODUCT_DEFINITION_FORMATION('',$,#7842);
#7838=APPLICATION_CONTEXT(
'Core Data for Automotive Mechanical Design Process');
#7839=PRODUCT_CONTEXT('part definition',#7838,'mechanical');
#7842=PRODUCT('Side plate','Side plate','Side plate',(#7839));
#7918=COLOUR_RGB('Sky Blue',0.24,0.69,0.87);
#7919=FILL_AREA_STYLE_COLOUR('',#7918);
#7920=FILL_AREA_STYLE('',(#7919));
#7921=SURFACE_STYLE_FILL_AREA(#7920);
#7922=SURFACE_SIDE_STYLE('',(#7921));
#7923=SURFACE_STYLE_USAGE(.BOTH.,#7922);
#7924=PRESENTATION_STYLE_ASSIGNMENT((#7923));
ENDSEC;
END-ISO-10303-21;
